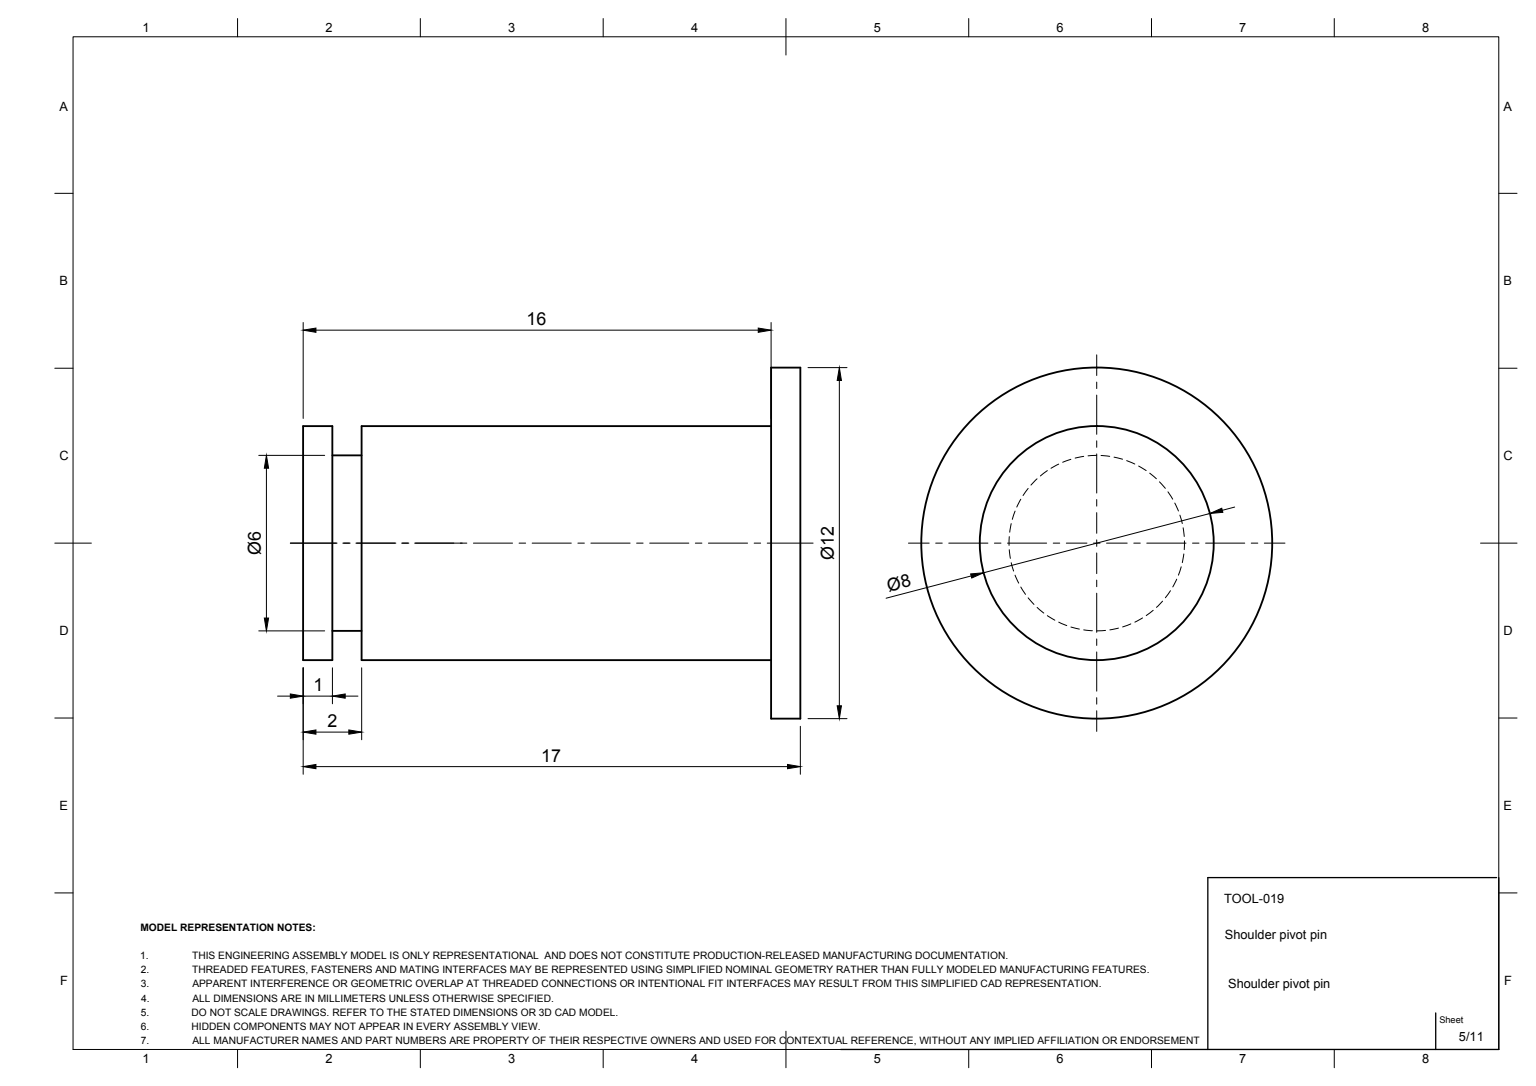
ISO-10303-21;
HEADER;
/* Generated by software containing ST-Developer
 * from STEP Tools, Inc. (www.steptools.com) 
 */

FILE_DESCRIPTION(
/* description */ (''),
/* implementation_level */ '2;1');

FILE_NAME(
/* name */ 'Shoulder pivot pin.step',
/* time_stamp */ '2026-11-10T09:14:46-08:00',
/* author */ (''),
/* organization */ (''),
/* preprocessor_version */ 'ST-DEVELOPER v20.2',
/* originating_system */ 'Autodesk Translation Framework v15.17.0.0',
/* authorisation */ '');

FILE_SCHEMA (('AUTOMOTIVE_DESIGN { 1 0 10303 214 3 1 1 }'));
ENDSEC;

DATA;
#10=MECHANICAL_DESIGN_GEOMETRIC_PRESENTATION_REPRESENTATION('',(#560),#19471);
#540=SHAPE_REPRESENTATION_RELATIONSHIP('SRR','None',#19519,#550);
#550=ADVANCED_BREP_SHAPE_REPRESENTATION('',(#570),#19462);
#560=STYLED_ITEM('',(#19582),#570);
#570=MANIFOLD_SOLID_BREP('Body1',#7153);
#598=FACE_BOUND('',#1315,.T.);
#599=FACE_BOUND('',#1317,.T.);
#600=FACE_BOUND('',#1320,.T.);
#697=PLANE('',#7397);
#698=PLANE('',#7399);
#699=PLANE('',#7403);
#700=PLANE('',#7408);
#701=PLANE('',#7410);
#888=FACE_OUTER_BOUND('',#1313,.T.);
#889=FACE_OUTER_BOUND('',#1314,.T.);
#890=FACE_OUTER_BOUND('',#1316,.T.);
#891=FACE_OUTER_BOUND('',#1318,.T.);
#892=FACE_OUTER_BOUND('',#1319,.T.);
#893=FACE_OUTER_BOUND('',#1321,.T.);
#894=FACE_OUTER_BOUND('',#1322,.T.);
#895=FACE_OUTER_BOUND('',#1323,.T.);
#896=FACE_OUTER_BOUND('',#1324,.T.);
#1313=EDGE_LOOP('',(#4901,#4902,#4903,#4904));
#1314=EDGE_LOOP('',(#4905));
#1315=EDGE_LOOP('',(#4906));
#1316=EDGE_LOOP('',(#4907));
#1317=EDGE_LOOP('',(#4908));
#1318=EDGE_LOOP('',(#4909,#4910,#4911,#4912));
#1319=EDGE_LOOP('',(#4913));
#1320=EDGE_LOOP('',(#4914));
#1321=EDGE_LOOP('',(#4915,#4916,#4917,#4918));
#1322=EDGE_LOOP('',(#4919));
#1323=EDGE_LOOP('',(#4920,#4921,#4922,#4923));
#1324=EDGE_LOOP('',(#4924));
#1839=LINE('',#9759,#2313);
#1840=LINE('',#9770,#2314);
#1841=LINE('',#9778,#2315);
#1842=LINE('',#9782,#2316);
#2313=VECTOR('',#8197,0.3);
#2314=VECTOR('',#8212,0.4);
#2315=VECTOR('',#8221,0.6);
#2316=VECTOR('',#8228,0.4);
#2707=CIRCLE('',#7395,0.3);
#2708=CIRCLE('',#7396,0.3);
#2709=CIRCLE('',#7398,0.4);
#2710=CIRCLE('',#7400,0.4);
#2711=CIRCLE('',#7402,0.4);
#2712=CIRCLE('',#7404,0.6);
#2713=CIRCLE('',#7405,0.4);
#2714=CIRCLE('',#7407,0.6);
#2963=VERTEX_POINT('',#9756);
#2964=VERTEX_POINT('',#9758);
#2965=VERTEX_POINT('',#9762);
#2966=VERTEX_POINT('',#9765);
#2967=VERTEX_POINT('',#9768);
#2968=VERTEX_POINT('',#9772);
#2969=VERTEX_POINT('',#9774);
#2970=VERTEX_POINT('',#9777);
#3691=EDGE_CURVE('',#2963,#2963,#2707,.T.);
#3692=EDGE_CURVE('',#2963,#2964,#1839,.T.);
#3693=EDGE_CURVE('',#2964,#2964,#2708,.T.);
#3694=EDGE_CURVE('',#2965,#2965,#2709,.T.);
#3695=EDGE_CURVE('',#2966,#2966,#2710,.T.);
#3696=EDGE_CURVE('',#2967,#2967,#2711,.T.);
#3697=EDGE_CURVE('',#2967,#2966,#1840,.T.);
#3698=EDGE_CURVE('',#2968,#2968,#2712,.T.);
#3699=EDGE_CURVE('',#2969,#2969,#2713,.T.);
#3700=EDGE_CURVE('',#2968,#2970,#1841,.T.);
#3701=EDGE_CURVE('',#2970,#2970,#2714,.T.);
#3702=EDGE_CURVE('',#2965,#2969,#1842,.T.);
#4901=ORIENTED_EDGE('',*,*,#3691,.T.);
#4902=ORIENTED_EDGE('',*,*,#3692,.T.);
#4903=ORIENTED_EDGE('',*,*,#3693,.F.);
#4904=ORIENTED_EDGE('',*,*,#3692,.F.);
#4905=ORIENTED_EDGE('',*,*,#3694,.F.);
#4906=ORIENTED_EDGE('',*,*,#3691,.F.);
#4907=ORIENTED_EDGE('',*,*,#3695,.F.);
#4908=ORIENTED_EDGE('',*,*,#3693,.T.);
#4909=ORIENTED_EDGE('',*,*,#3696,.F.);
#4910=ORIENTED_EDGE('',*,*,#3697,.T.);
#4911=ORIENTED_EDGE('',*,*,#3695,.T.);
#4912=ORIENTED_EDGE('',*,*,#3697,.F.);
#4913=ORIENTED_EDGE('',*,*,#3698,.T.);
#4914=ORIENTED_EDGE('',*,*,#3699,.F.);
#4915=ORIENTED_EDGE('',*,*,#3698,.F.);
#4916=ORIENTED_EDGE('',*,*,#3700,.T.);
#4917=ORIENTED_EDGE('',*,*,#3701,.T.);
#4918=ORIENTED_EDGE('',*,*,#3700,.F.);
#4919=ORIENTED_EDGE('',*,*,#3701,.F.);
#4920=ORIENTED_EDGE('',*,*,#3694,.T.);
#4921=ORIENTED_EDGE('',*,*,#3702,.T.);
#4922=ORIENTED_EDGE('',*,*,#3699,.T.);
#4923=ORIENTED_EDGE('',*,*,#3702,.F.);
#4924=ORIENTED_EDGE('',*,*,#3696,.T.);
#6621=CYLINDRICAL_SURFACE('',#7394,0.3);
#6622=CYLINDRICAL_SURFACE('',#7401,0.4);
#6623=CYLINDRICAL_SURFACE('',#7406,0.6);
#6624=CYLINDRICAL_SURFACE('',#7409,0.4);
#6810=ADVANCED_FACE('',(#888),#6621,.T.);
#6811=ADVANCED_FACE('',(#889,#598),#697,.F.);
#6812=ADVANCED_FACE('',(#890,#599),#698,.F.);
#6813=ADVANCED_FACE('',(#891),#6622,.T.);
#6814=ADVANCED_FACE('',(#892,#600),#699,.T.);
#6815=ADVANCED_FACE('',(#893),#6623,.T.);
#6816=ADVANCED_FACE('',(#894),#700,.F.);
#6817=ADVANCED_FACE('',(#895),#6624,.T.);
#6818=ADVANCED_FACE('',(#896),#701,.T.);
#7153=CLOSED_SHELL('',(#6810,#6811,#6812,#6813,#6814,#6815,#6816,#6817,
#6818));
#7393=AXIS2_PLACEMENT_3D('',#9754,#8191,#8192);
#7394=AXIS2_PLACEMENT_3D('',#9755,#8193,#8194);
#7395=AXIS2_PLACEMENT_3D('',#9757,#8195,#8196);
#7396=AXIS2_PLACEMENT_3D('',#9760,#8198,#8199);
#7397=AXIS2_PLACEMENT_3D('',#9761,#8200,#8201);
#7398=AXIS2_PLACEMENT_3D('',#9763,#8202,#8203);
#7399=AXIS2_PLACEMENT_3D('',#9764,#8204,#8205);
#7400=AXIS2_PLACEMENT_3D('',#9766,#8206,#8207);
#7401=AXIS2_PLACEMENT_3D('',#9767,#8208,#8209);
#7402=AXIS2_PLACEMENT_3D('',#9769,#8210,#8211);
#7403=AXIS2_PLACEMENT_3D('',#9771,#8213,#8214);
#7404=AXIS2_PLACEMENT_3D('',#9773,#8215,#8216);
#7405=AXIS2_PLACEMENT_3D('',#9775,#8217,#8218);
#7406=AXIS2_PLACEMENT_3D('',#9776,#8219,#8220);
#7407=AXIS2_PLACEMENT_3D('',#9779,#8222,#8223);
#7408=AXIS2_PLACEMENT_3D('',#9780,#8224,#8225);
#7409=AXIS2_PLACEMENT_3D('',#9781,#8226,#8227);
#7410=AXIS2_PLACEMENT_3D('',#9783,#8229,#8230);
#8191=DIRECTION('axis',(0.,0.,1.));
#8192=DIRECTION('refdir',(1.,0.,0.));
#8193=DIRECTION('center_axis',(0.,0.,1.));
#8194=DIRECTION('ref_axis',(1.,0.,0.));
#8195=DIRECTION('center_axis',(0.,0.,1.));
#8196=DIRECTION('ref_axis',(1.,0.,0.));
#8197=DIRECTION('',(0.,0.,1.));
#8198=DIRECTION('center_axis',(0.,0.,1.));
#8199=DIRECTION('ref_axis',(1.,0.,0.));
#8200=DIRECTION('center_axis',(0.,0.,-1.));
#8201=DIRECTION('ref_axis',(-1.,0.,0.));
#8202=DIRECTION('center_axis',(0.,0.,-1.));
#8203=DIRECTION('ref_axis',(1.,0.,0.));
#8204=DIRECTION('center_axis',(0.,0.,1.));
#8205=DIRECTION('ref_axis',(1.,0.,0.));
#8206=DIRECTION('center_axis',(0.,0.,1.));
#8207=DIRECTION('ref_axis',(1.,0.,0.));
#8208=DIRECTION('center_axis',(0.,0.,1.));
#8209=DIRECTION('ref_axis',(1.,0.,0.));
#8210=DIRECTION('center_axis',(0.,0.,1.));
#8211=DIRECTION('ref_axis',(1.,0.,0.));
#8212=DIRECTION('',(0.,0.,-1.));
#8213=DIRECTION('center_axis',(0.,0.,1.));
#8214=DIRECTION('ref_axis',(1.,0.,0.));
#8215=DIRECTION('center_axis',(0.,0.,1.));
#8216=DIRECTION('ref_axis',(1.,0.,0.));
#8217=DIRECTION('center_axis',(0.,0.,1.));
#8218=DIRECTION('ref_axis',(1.,0.,0.));
#8219=DIRECTION('center_axis',(0.,0.,1.));
#8220=DIRECTION('ref_axis',(1.,0.,0.));
#8221=DIRECTION('',(0.,0.,-1.));
#8222=DIRECTION('center_axis',(0.,0.,1.));
#8223=DIRECTION('ref_axis',(1.,0.,0.));
#8224=DIRECTION('center_axis',(0.,0.,1.));
#8225=DIRECTION('ref_axis',(1.,0.,0.));
#8226=DIRECTION('center_axis',(0.,0.,1.));
#8227=DIRECTION('ref_axis',(1.,0.,0.));
#8228=DIRECTION('',(0.,0.,-1.));
#8229=DIRECTION('center_axis',(0.,0.,1.));
#8230=DIRECTION('ref_axis',(1.,0.,0.));
#9754=CARTESIAN_POINT('',(0.,0.,0.));
#9755=CARTESIAN_POINT('Origin',(0.,0.,0.75));
#9756=CARTESIAN_POINT('',(-0.3,-3.67394039744206E-17,0.7));
#9757=CARTESIAN_POINT('Origin',(0.,0.,0.7));
#9758=CARTESIAN_POINT('',(-0.3,-3.67394039744206E-17,0.8));
#9759=CARTESIAN_POINT('',(-0.3,-3.67394039744206E-17,0.75));
#9760=CARTESIAN_POINT('Origin',(0.,0.,0.8));
#9761=CARTESIAN_POINT('Origin',(0.7,0.,0.7));
#9762=CARTESIAN_POINT('',(-0.4,4.89858719658941E-17,0.7));
#9763=CARTESIAN_POINT('Origin',(0.,0.,0.7));
#9764=CARTESIAN_POINT('Origin',(0.3,0.,0.8));
#9765=CARTESIAN_POINT('',(-0.4,-4.89858719658941E-17,0.8));
#9766=CARTESIAN_POINT('Origin',(0.,0.,0.8));
#9767=CARTESIAN_POINT('Origin',(0.,0.,-0.7));
#9768=CARTESIAN_POINT('',(-0.4,-4.89858719658941E-17,0.9));
#9769=CARTESIAN_POINT('Origin',(0.,0.,0.9));
#9770=CARTESIAN_POINT('',(-0.4,-4.89858719658941E-17,-0.7));
#9771=CARTESIAN_POINT('Origin',(0.,0.,-0.7));
#9772=CARTESIAN_POINT('',(-0.6,-7.34788079488412E-17,-0.7));
#9773=CARTESIAN_POINT('Origin',(0.,0.,-0.7));
#9774=CARTESIAN_POINT('',(-0.4,-4.89858719658941E-17,-0.7));
#9775=CARTESIAN_POINT('Origin',(0.,0.,-0.7));
#9776=CARTESIAN_POINT('Origin',(0.,0.,-0.8));
#9777=CARTESIAN_POINT('',(-0.6,-7.34788079488412E-17,-0.8));
#9778=CARTESIAN_POINT('',(-0.6,-7.34788079488412E-17,-0.8));
#9779=CARTESIAN_POINT('Origin',(0.,0.,-0.8));
#9780=CARTESIAN_POINT('Origin',(0.,0.,-0.8));
#9781=CARTESIAN_POINT('Origin',(0.,0.,-0.7));
#9782=CARTESIAN_POINT('',(-0.4,-4.89858719658941E-17,-0.7));
#9783=CARTESIAN_POINT('Origin',(0.,0.,0.9));
#19449=UNCERTAINTY_MEASURE_WITH_UNIT(LENGTH_MEASURE(0.001),#19472,
'DISTANCE_ACCURACY_VALUE',
'Maximum model space distance between geometric entities at asserted c
onnectivities');
#19458=UNCERTAINTY_MEASURE_WITH_UNIT(LENGTH_MEASURE(0.001),#19472,
'DISTANCE_ACCURACY_VALUE',
'Maximum model space distance between geometric entities at asserted c
onnectivities');
#19462=(
GEOMETRIC_REPRESENTATION_CONTEXT(3)
GLOBAL_UNCERTAINTY_ASSIGNED_CONTEXT((#19449))
GLOBAL_UNIT_ASSIGNED_CONTEXT((#19472,#19474,#19475))
REPRESENTATION_CONTEXT('','3D')
);
#19471=(
GEOMETRIC_REPRESENTATION_CONTEXT(3)
GLOBAL_UNCERTAINTY_ASSIGNED_CONTEXT((#19458))
GLOBAL_UNIT_ASSIGNED_CONTEXT((#19472,#19474,#19475))
REPRESENTATION_CONTEXT('','3D')
);
#19472=(
LENGTH_UNIT()
NAMED_UNIT(*)
SI_UNIT(.CENTI.,.METRE.)
);
#19474=(
NAMED_UNIT(*)
PLANE_ANGLE_UNIT()
SI_UNIT($,.RADIAN.)
);
#19475=(
NAMED_UNIT(*)
SI_UNIT($,.STERADIAN.)
SOLID_ANGLE_UNIT()
);
#19479=SHAPE_DEFINITION_REPRESENTATION(#19491,#19519);
#19491=PRODUCT_DEFINITION_SHAPE('',$,#19532);
#19519=SHAPE_REPRESENTATION('',(#7393),#19462);
#19528=PRODUCT_DEFINITION_CONTEXT('part definition',#19566,'design');
#19532=PRODUCT_DEFINITION('Shoulder pivot pin','Shoulder pivot pin',#19544,
#19528);
#19544=PRODUCT_DEFINITION_FORMATION('',$,#19571);
#19566=APPLICATION_CONTEXT(
'Core Data for Automotive Mechanical Design Process');
#19567=PRODUCT_CONTEXT('part definition',#19566,'mechanical');
#19571=PRODUCT('Shoulder pivot pin','Shoulder pivot pin',$,(#19567));
#19582=PRESENTATION_STYLE_ASSIGNMENT((#19590));
#19590=SURFACE_STYLE_USAGE(.BOTH.,#19598);
#19598=SURFACE_SIDE_STYLE('',(#19606));
#19606=SURFACE_STYLE_FILL_AREA(#19614);
#19614=FILL_AREA_STYLE('Pivot dark gray',(#19622));
#19622=FILL_AREA_STYLE_COLOUR('Pivot dark gray',#19630);
#19630=COLOUR_RGB('Pivot dark gray',0.27843137254902,0.309803921568627,
0.352941176470588);
ENDSEC;
END-ISO-10303-21;
